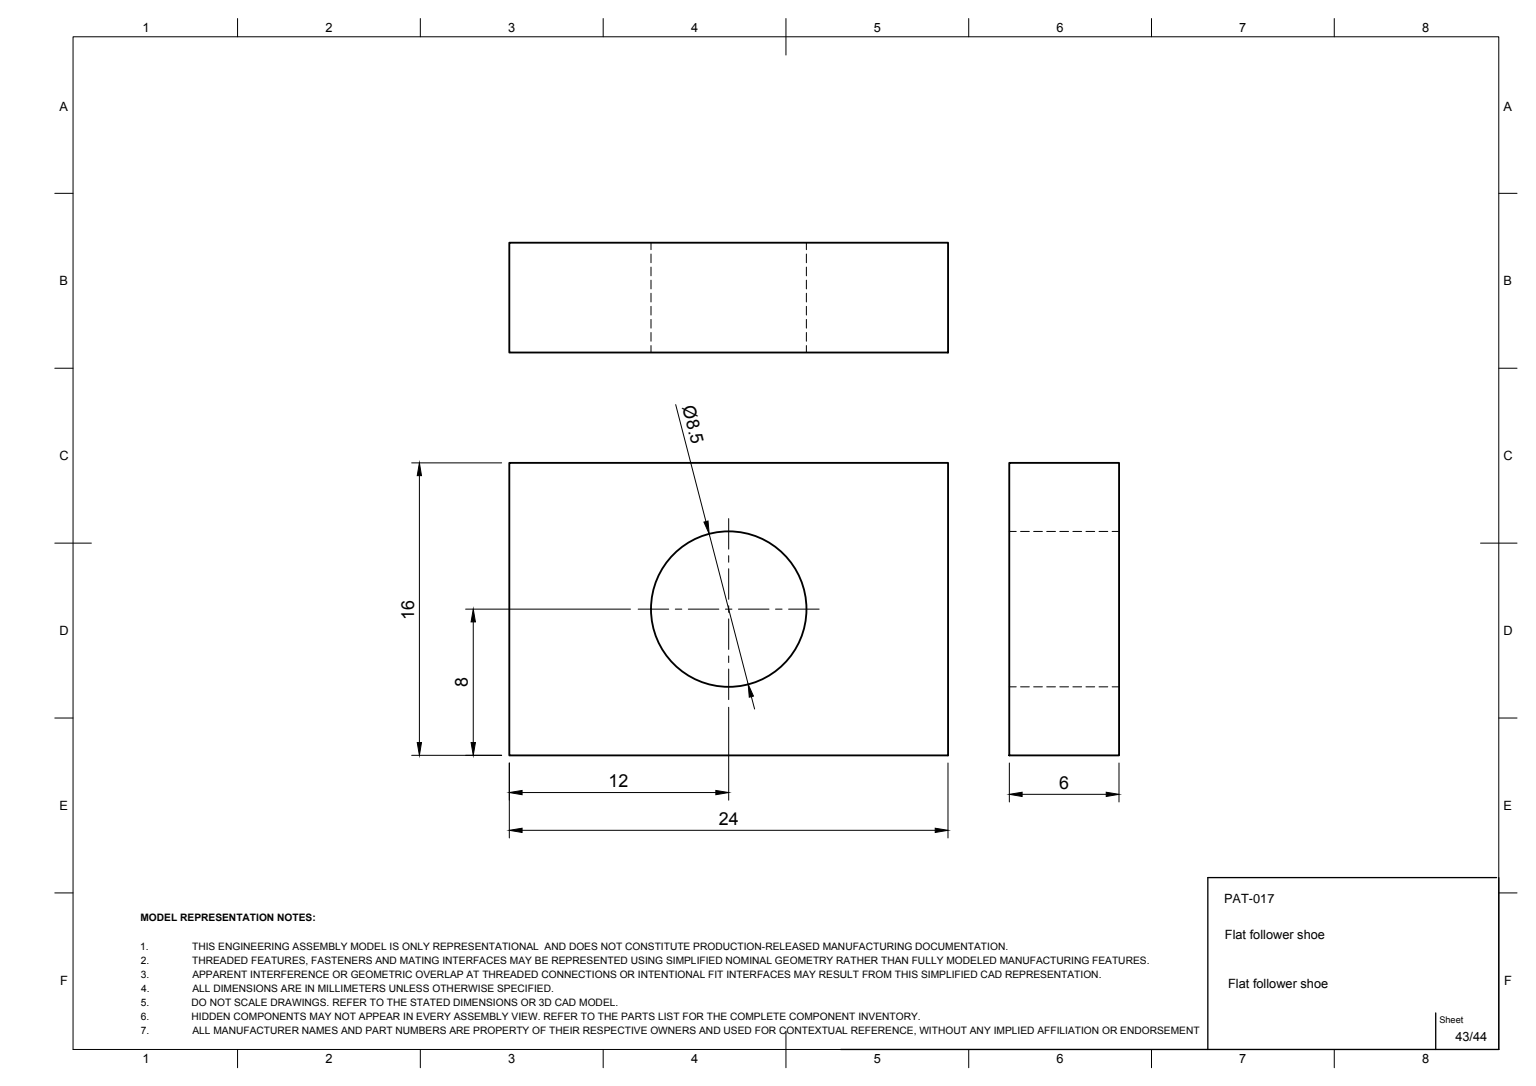
ISO-10303-21;
HEADER;
/* Generated by software containing ST-Developer
 * from STEP Tools, Inc. (www.steptools.com) 
 */

FILE_DESCRIPTION(
/* description */ ('Cam-and-follower valve demonstrator'),
/* implementation_level */ '2;1');

FILE_NAME(
/* name */ 'Flat follower shoe.step',
/* time_stamp */ '2026-10-28T03:25:17-07:00',
/* author */ (''),
/* organization */ (''),
/* preprocessor_version */ 'ST-DEVELOPER v20.2',
/* originating_system */ 'Autodesk Translation Framework v15.17.0.0',
/* authorisation */ '');

FILE_SCHEMA (('AUTOMOTIVE_DESIGN { 1 0 10303 214 3 1 1 }'));
ENDSEC;

DATA;
#10=MECHANICAL_DESIGN_GEOMETRIC_PRESENTATION_REPRESENTATION('',(#452),#12896);
#373=SHAPE_REPRESENTATION_RELATIONSHIP('SRR','None',#13093,#409);
#409=ADVANCED_BREP_SHAPE_REPRESENTATION('',(#492),#12893);
#452=STYLED_ITEM('',(#13316),#492);
#492=MANIFOLD_SOLID_BREP('Body1',#6222);
#653=FACE_BOUND('',#1977,.T.);
#654=FACE_BOUND('',#1979,.T.);
#961=CIRCLE('',#7377,0.425);
#962=CIRCLE('',#7378,0.425);
#1089=CYLINDRICAL_SURFACE('',#7376,0.425);
#1445=FACE_OUTER_BOUND('',#1971,.T.);
#1446=FACE_OUTER_BOUND('',#1972,.T.);
#1447=FACE_OUTER_BOUND('',#1973,.T.);
#1448=FACE_OUTER_BOUND('',#1974,.T.);
#1449=FACE_OUTER_BOUND('',#1975,.T.);
#1450=FACE_OUTER_BOUND('',#1976,.T.);
#1451=FACE_OUTER_BOUND('',#1978,.T.);
#1971=EDGE_LOOP('',(#5537,#5538,#5539,#5540));
#1972=EDGE_LOOP('',(#5541,#5542,#5543,#5544));
#1973=EDGE_LOOP('',(#5545,#5546,#5547,#5548));
#1974=EDGE_LOOP('',(#5549,#5550,#5551,#5552));
#1975=EDGE_LOOP('',(#5553,#5554,#5555,#5556));
#1976=EDGE_LOOP('',(#5557,#5558,#5559,#5560));
#1977=EDGE_LOOP('',(#5561));
#1978=EDGE_LOOP('',(#5562,#5563,#5564,#5565));
#1979=EDGE_LOOP('',(#5566));
#2399=LINE('',#12739,#2821);
#2400=LINE('',#12744,#2822);
#2401=LINE('',#12746,#2823);
#2402=LINE('',#12748,#2824);
#2403=LINE('',#12749,#2825);
#2404=LINE('',#12752,#2826);
#2405=LINE('',#12754,#2827);
#2406=LINE('',#12755,#2828);
#2407=LINE('',#12758,#2829);
#2408=LINE('',#12760,#2830);
#2409=LINE('',#12761,#2831);
#2410=LINE('',#12763,#2832);
#2411=LINE('',#12764,#2833);
#2821=VECTOR('',#9330,0.425);
#2822=VECTOR('',#9335,1.);
#2823=VECTOR('',#9336,1.);
#2824=VECTOR('',#9337,1.);
#2825=VECTOR('',#9338,1.);
#2826=VECTOR('',#9341,1.);
#2827=VECTOR('',#9342,1.);
#2828=VECTOR('',#9343,1.);
#2829=VECTOR('',#9346,1.);
#2830=VECTOR('',#9347,1.);
#2831=VECTOR('',#9348,1.);
#2832=VECTOR('',#9351,1.);
#2833=VECTOR('',#9352,1.);
#3324=VERTEX_POINT('',#12736);
#3325=VERTEX_POINT('',#12738);
#3326=VERTEX_POINT('',#12742);
#3327=VERTEX_POINT('',#12743);
#3328=VERTEX_POINT('',#12745);
#3329=VERTEX_POINT('',#12747);
#3330=VERTEX_POINT('',#12751);
#3331=VERTEX_POINT('',#12753);
#3332=VERTEX_POINT('',#12757);
#3333=VERTEX_POINT('',#12759);
#4065=EDGE_CURVE('',#3324,#3324,#961,.T.);
#4066=EDGE_CURVE('',#3324,#3325,#2399,.T.);
#4067=EDGE_CURVE('',#3325,#3325,#962,.T.);
#4068=EDGE_CURVE('',#3326,#3327,#2400,.T.);
#4069=EDGE_CURVE('',#3327,#3328,#2401,.T.);
#4070=EDGE_CURVE('',#3329,#3328,#2402,.T.);
#4071=EDGE_CURVE('',#3326,#3329,#2403,.T.);
#4072=EDGE_CURVE('',#3330,#3326,#2404,.T.);
#4073=EDGE_CURVE('',#3331,#3329,#2405,.T.);
#4074=EDGE_CURVE('',#3330,#3331,#2406,.T.);
#4075=EDGE_CURVE('',#3332,#3330,#2407,.T.);
#4076=EDGE_CURVE('',#3333,#3331,#2408,.T.);
#4077=EDGE_CURVE('',#3332,#3333,#2409,.T.);
#4078=EDGE_CURVE('',#3327,#3332,#2410,.T.);
#4079=EDGE_CURVE('',#3328,#3333,#2411,.T.);
#5537=ORIENTED_EDGE('',*,*,#4065,.F.);
#5538=ORIENTED_EDGE('',*,*,#4066,.T.);
#5539=ORIENTED_EDGE('',*,*,#4067,.F.);
#5540=ORIENTED_EDGE('',*,*,#4066,.F.);
#5541=ORIENTED_EDGE('',*,*,#4068,.T.);
#5542=ORIENTED_EDGE('',*,*,#4069,.T.);
#5543=ORIENTED_EDGE('',*,*,#4070,.F.);
#5544=ORIENTED_EDGE('',*,*,#4071,.F.);
#5545=ORIENTED_EDGE('',*,*,#4072,.T.);
#5546=ORIENTED_EDGE('',*,*,#4071,.T.);
#5547=ORIENTED_EDGE('',*,*,#4073,.F.);
#5548=ORIENTED_EDGE('',*,*,#4074,.F.);
#5549=ORIENTED_EDGE('',*,*,#4075,.T.);
#5550=ORIENTED_EDGE('',*,*,#4074,.T.);
#5551=ORIENTED_EDGE('',*,*,#4076,.F.);
#5552=ORIENTED_EDGE('',*,*,#4077,.F.);
#5553=ORIENTED_EDGE('',*,*,#4078,.T.);
#5554=ORIENTED_EDGE('',*,*,#4077,.T.);
#5555=ORIENTED_EDGE('',*,*,#4079,.F.);
#5556=ORIENTED_EDGE('',*,*,#4069,.F.);
#5557=ORIENTED_EDGE('',*,*,#4079,.T.);
#5558=ORIENTED_EDGE('',*,*,#4076,.T.);
#5559=ORIENTED_EDGE('',*,*,#4073,.T.);
#5560=ORIENTED_EDGE('',*,*,#4070,.T.);
#5561=ORIENTED_EDGE('',*,*,#4067,.T.);
#5562=ORIENTED_EDGE('',*,*,#4078,.F.);
#5563=ORIENTED_EDGE('',*,*,#4068,.F.);
#5564=ORIENTED_EDGE('',*,*,#4072,.F.);
#5565=ORIENTED_EDGE('',*,*,#4075,.F.);
#5566=ORIENTED_EDGE('',*,*,#4065,.T.);
#5799=PLANE('',#7379);
#5800=PLANE('',#7380);
#5801=PLANE('',#7381);
#5802=PLANE('',#7382);
#5803=PLANE('',#7383);
#5804=PLANE('',#7384);
#6161=ADVANCED_FACE('',(#1445),#1089,.F.);
#6162=ADVANCED_FACE('',(#1446),#5799,.T.);
#6163=ADVANCED_FACE('',(#1447),#5800,.T.);
#6164=ADVANCED_FACE('',(#1448),#5801,.T.);
#6165=ADVANCED_FACE('',(#1449),#5802,.T.);
#6166=ADVANCED_FACE('',(#1450,#653),#5803,.T.);
#6167=ADVANCED_FACE('',(#1451,#654),#5804,.F.);
#6222=CLOSED_SHELL('',(#6161,#6162,#6163,#6164,#6165,#6166,#6167));
#7375=AXIS2_PLACEMENT_3D('',#12734,#9324,#9325);
#7376=AXIS2_PLACEMENT_3D('',#12735,#9326,#9327);
#7377=AXIS2_PLACEMENT_3D('',#12737,#9328,#9329);
#7378=AXIS2_PLACEMENT_3D('',#12740,#9331,#9332);
#7379=AXIS2_PLACEMENT_3D('',#12741,#9333,#9334);
#7380=AXIS2_PLACEMENT_3D('',#12750,#9339,#9340);
#7381=AXIS2_PLACEMENT_3D('',#12756,#9344,#9345);
#7382=AXIS2_PLACEMENT_3D('',#12762,#9349,#9350);
#7383=AXIS2_PLACEMENT_3D('',#12765,#9353,#9354);
#7384=AXIS2_PLACEMENT_3D('',#12766,#9355,#9356);
#9324=DIRECTION('axis',(0.,0.,1.));
#9325=DIRECTION('refdir',(1.,0.,0.));
#9326=DIRECTION('center_axis',(0.,0.,1.));
#9327=DIRECTION('ref_axis',(1.,0.,0.));
#9328=DIRECTION('center_axis',(0.,0.,1.));
#9329=DIRECTION('ref_axis',(1.,0.,0.));
#9330=DIRECTION('',(0.,0.,1.));
#9331=DIRECTION('center_axis',(0.,0.,-1.));
#9332=DIRECTION('ref_axis',(1.,0.,0.));
#9333=DIRECTION('center_axis',(0.,1.,0.));
#9334=DIRECTION('ref_axis',(-1.,0.,0.));
#9335=DIRECTION('',(-1.,0.,0.));
#9336=DIRECTION('',(0.,0.,1.));
#9337=DIRECTION('',(-1.,0.,0.));
#9338=DIRECTION('',(0.,0.,1.));
#9339=DIRECTION('center_axis',(1.,0.,0.));
#9340=DIRECTION('ref_axis',(0.,1.,0.));
#9341=DIRECTION('',(0.,1.,0.));
#9342=DIRECTION('',(0.,1.,0.));
#9343=DIRECTION('',(0.,0.,1.));
#9344=DIRECTION('center_axis',(0.,-1.,0.));
#9345=DIRECTION('ref_axis',(1.,0.,0.));
#9346=DIRECTION('',(1.,0.,0.));
#9347=DIRECTION('',(1.,0.,0.));
#9348=DIRECTION('',(0.,0.,1.));
#9349=DIRECTION('center_axis',(-1.,0.,0.));
#9350=DIRECTION('ref_axis',(0.,-1.,0.));
#9351=DIRECTION('',(0.,-1.,0.));
#9352=DIRECTION('',(0.,-1.,0.));
#9353=DIRECTION('center_axis',(0.,0.,1.));
#9354=DIRECTION('ref_axis',(1.,0.,0.));
#9355=DIRECTION('center_axis',(0.,0.,1.));
#9356=DIRECTION('ref_axis',(1.,0.,0.));
#12734=CARTESIAN_POINT('',(0.,0.,0.));
#12735=CARTESIAN_POINT('Origin',(0.,0.,6.3));
#12736=CARTESIAN_POINT('',(-0.425,-5.20474889637625E-17,6.4));
#12737=CARTESIAN_POINT('Origin',(0.,0.,6.4));
#12738=CARTESIAN_POINT('',(-0.425,5.20474889637625E-17,7.));
#12739=CARTESIAN_POINT('',(-0.425,-5.20474889637625E-17,6.3));
#12740=CARTESIAN_POINT('Origin',(0.,0.,7.));
#12741=CARTESIAN_POINT('Origin',(1.2,0.8,6.4));
#12742=CARTESIAN_POINT('',(1.2,0.8,6.4));
#12743=CARTESIAN_POINT('',(-1.2,0.8,6.4));
#12744=CARTESIAN_POINT('',(1.2,0.8,6.4));
#12745=CARTESIAN_POINT('',(-1.2,0.8,7.));
#12746=CARTESIAN_POINT('',(-1.2,0.8,6.4));
#12747=CARTESIAN_POINT('',(1.2,0.8,7.));
#12748=CARTESIAN_POINT('',(1.2,0.8,7.));
#12749=CARTESIAN_POINT('',(1.2,0.8,6.4));
#12750=CARTESIAN_POINT('Origin',(1.2,-0.8,6.4));
#12751=CARTESIAN_POINT('',(1.2,-0.8,6.4));
#12752=CARTESIAN_POINT('',(1.2,-0.8,6.4));
#12753=CARTESIAN_POINT('',(1.2,-0.8,7.));
#12754=CARTESIAN_POINT('',(1.2,-0.8,7.));
#12755=CARTESIAN_POINT('',(1.2,-0.8,6.4));
#12756=CARTESIAN_POINT('Origin',(-1.2,-0.8,6.4));
#12757=CARTESIAN_POINT('',(-1.2,-0.8,6.4));
#12758=CARTESIAN_POINT('',(-1.2,-0.8,6.4));
#12759=CARTESIAN_POINT('',(-1.2,-0.8,7.));
#12760=CARTESIAN_POINT('',(-1.2,-0.8,7.));
#12761=CARTESIAN_POINT('',(-1.2,-0.8,6.4));
#12762=CARTESIAN_POINT('Origin',(-1.2,0.8,6.4));
#12763=CARTESIAN_POINT('',(-1.2,0.8,6.4));
#12764=CARTESIAN_POINT('',(-1.2,0.8,7.));
#12765=CARTESIAN_POINT('Origin',(0.,0.,7.));
#12766=CARTESIAN_POINT('Origin',(0.,0.,6.4));
#12850=UNCERTAINTY_MEASURE_WITH_UNIT(LENGTH_MEASURE(0.001),#12897,
'DISTANCE_ACCURACY_VALUE',
'Maximum model space distance between geometric entities at asserted c
onnectivities');
#12853=UNCERTAINTY_MEASURE_WITH_UNIT(LENGTH_MEASURE(0.001),#12897,
'DISTANCE_ACCURACY_VALUE',
'Maximum model space distance between geometric entities at asserted c
onnectivities');
#12893=(
GEOMETRIC_REPRESENTATION_CONTEXT(3)
GLOBAL_UNCERTAINTY_ASSIGNED_CONTEXT((#12850))
GLOBAL_UNIT_ASSIGNED_CONTEXT((#12897,#12899,#12900))
REPRESENTATION_CONTEXT('','3D')
);
#12896=(
GEOMETRIC_REPRESENTATION_CONTEXT(3)
GLOBAL_UNCERTAINTY_ASSIGNED_CONTEXT((#12853))
GLOBAL_UNIT_ASSIGNED_CONTEXT((#12897,#12899,#12900))
REPRESENTATION_CONTEXT('','3D')
);
#12897=(
LENGTH_UNIT()
NAMED_UNIT(*)
SI_UNIT(.CENTI.,.METRE.)
);
#12899=(
NAMED_UNIT(*)
PLANE_ANGLE_UNIT()
SI_UNIT($,.RADIAN.)
);
#12900=(
NAMED_UNIT(*)
SI_UNIT($,.STERADIAN.)
SOLID_ANGLE_UNIT()
);
#12940=SHAPE_DEFINITION_REPRESENTATION(#13045,#13093);
#13045=PRODUCT_DEFINITION_SHAPE('',$,#13136);
#13093=SHAPE_REPRESENTATION('',(#7375),#12893);
#13096=PRODUCT_DEFINITION_CONTEXT('part definition',#13224,'design');
#13136=PRODUCT_DEFINITION('Flat follower shoe','Flat follower shoe',#13178,
#13096);
#13178=PRODUCT_DEFINITION_FORMATION('',$,#13265);
#13224=APPLICATION_CONTEXT(
'Core Data for Automotive Mechanical Design Process');
#13225=PRODUCT_CONTEXT('part definition',#13224,'mechanical');
#13265=PRODUCT('Flat follower shoe','Flat follower shoe',
'Flat follower shoe',(#13225));
#13310=COLOUR_RGB('Light Blue',0.38,0.62,0.78);
#13311=FILL_AREA_STYLE_COLOUR('',#13310);
#13312=FILL_AREA_STYLE('',(#13311));
#13313=SURFACE_STYLE_FILL_AREA(#13312);
#13314=SURFACE_SIDE_STYLE('',(#13313));
#13315=SURFACE_STYLE_USAGE(.BOTH.,#13314);
#13316=PRESENTATION_STYLE_ASSIGNMENT((#13315));
ENDSEC;
END-ISO-10303-21;
